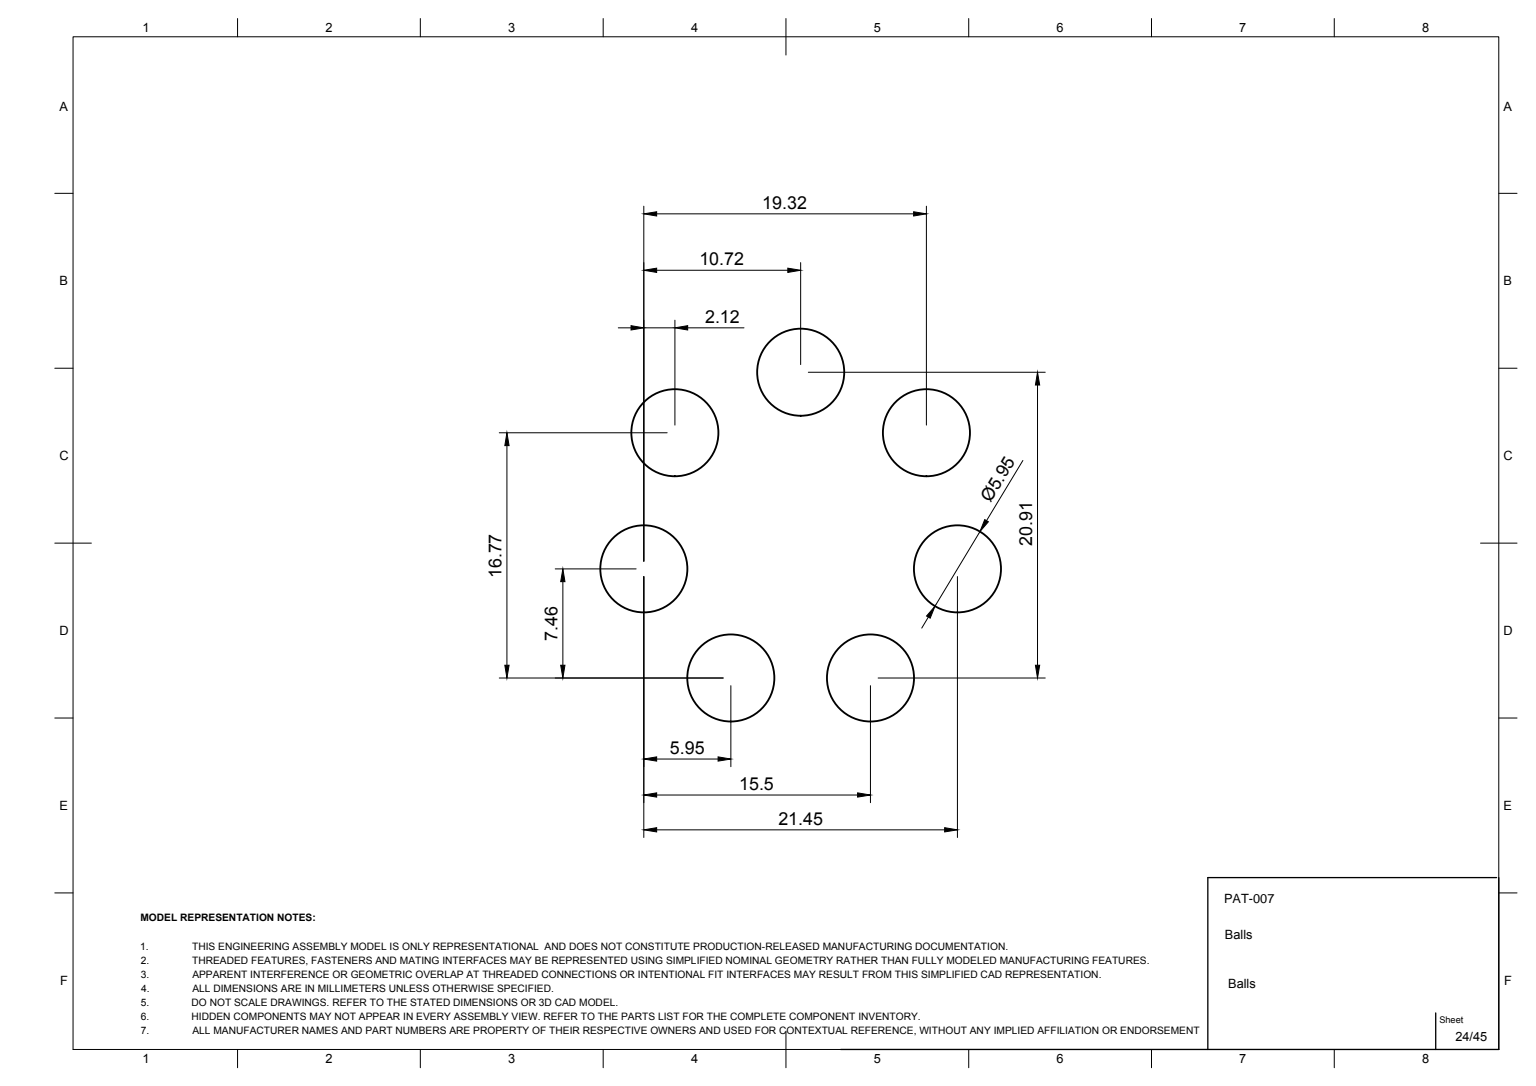
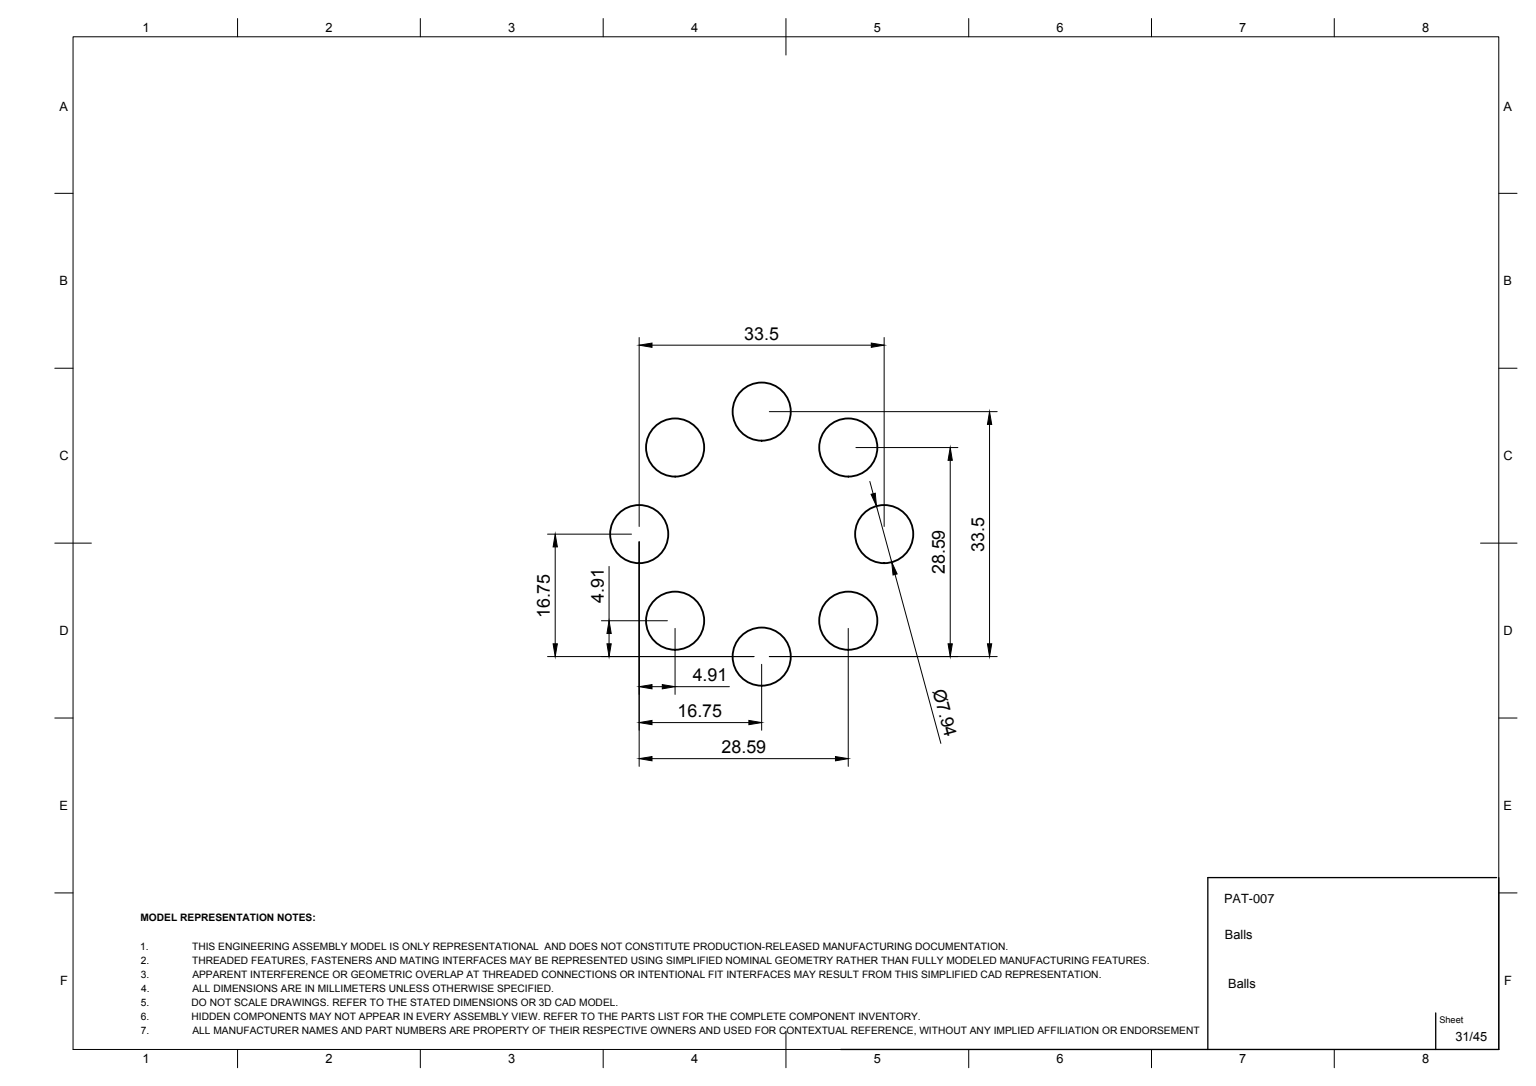
ISO-10303-21;
HEADER;
/* Generated by software containing ST-Developer
 * from STEP Tools, Inc. (www.steptools.com) 
 */

FILE_DESCRIPTION(
/* description */ ('Bearing friction torque test rig'),
/* implementation_level */ '2;1');

FILE_NAME(
/* name */ 'Balls.step',
/* time_stamp */ '2026-10-28T03:24:04-07:00',
/* author */ (''),
/* organization */ (''),
/* preprocessor_version */ 'ST-DEVELOPER v20.2',
/* originating_system */ 'Autodesk Translation Framework v15.17.0.0',
/* authorisation */ '');

FILE_SCHEMA (('AUTOMOTIVE_DESIGN { 1 0 10303 214 3 1 1 }'));
ENDSEC;

DATA;
#10=MECHANICAL_DESIGN_GEOMETRIC_PRESENTATION_REPRESENTATION('',(#557,#558,#559,#560,#561,#562,#563),#14822);
#395=SPHERICAL_SURFACE('',#8664,0.29765);
#396=SPHERICAL_SURFACE('',#8666,0.29765);
#397=SPHERICAL_SURFACE('',#8668,0.29765);
#398=SPHERICAL_SURFACE('',#8670,0.29765);
#399=SPHERICAL_SURFACE('',#8672,0.29765);
#400=SPHERICAL_SURFACE('',#8674,0.29765);
#401=SPHERICAL_SURFACE('',#8676,0.29765);
#479=SHAPE_REPRESENTATION_RELATIONSHIP('SRR','None',#15019,#518);
#518=ADVANCED_BREP_SHAPE_REPRESENTATION('',(#610,#611,#612,#613,#614,#615,
#616),#14799);
#557=STYLED_ITEM('',(#15284),#610);
#558=STYLED_ITEM('',(#15284),#611);
#559=STYLED_ITEM('',(#15284),#612);
#560=STYLED_ITEM('',(#15284),#613);
#561=STYLED_ITEM('',(#15284),#614);
#562=STYLED_ITEM('',(#15284),#615);
#563=STYLED_ITEM('',(#15284),#616);
#610=MANIFOLD_SOLID_BREP('Body1',#7674);
#611=MANIFOLD_SOLID_BREP('Body2',#7675);
#612=MANIFOLD_SOLID_BREP('Body3',#7676);
#613=MANIFOLD_SOLID_BREP('Body4',#7677);
#614=MANIFOLD_SOLID_BREP('Body5',#7678);
#615=MANIFOLD_SOLID_BREP('Body6',#7679);
#616=MANIFOLD_SOLID_BREP('Body7',#7680);
#1352=FACE_OUTER_BOUND('',#1971,.T.);
#1353=FACE_OUTER_BOUND('',#1972,.T.);
#1354=FACE_OUTER_BOUND('',#1973,.T.);
#1355=FACE_OUTER_BOUND('',#1974,.T.);
#1356=FACE_OUTER_BOUND('',#1975,.T.);
#1357=FACE_OUTER_BOUND('',#1976,.T.);
#1358=FACE_OUTER_BOUND('',#1977,.T.);
#1971=EDGE_LOOP('',(#6268,#6269));
#1972=EDGE_LOOP('',(#6270,#6271));
#1973=EDGE_LOOP('',(#6272,#6273));
#1974=EDGE_LOOP('',(#6274,#6275));
#1975=EDGE_LOOP('',(#6276,#6277));
#1976=EDGE_LOOP('',(#6278,#6279));
#1977=EDGE_LOOP('',(#6280,#6281));
#3348=CIRCLE('',#8665,0.29765);
#3349=CIRCLE('',#8667,0.29765);
#3350=CIRCLE('',#8669,0.29765);
#3351=CIRCLE('',#8671,0.29765);
#3352=CIRCLE('',#8673,0.29765);
#3353=CIRCLE('',#8675,0.29765);
#3354=CIRCLE('',#8677,0.29765);
#3924=VERTEX_POINT('',#12865);
#3925=VERTEX_POINT('',#12866);
#3926=VERTEX_POINT('',#12869);
#3927=VERTEX_POINT('',#12870);
#3928=VERTEX_POINT('',#12873);
#3929=VERTEX_POINT('',#12874);
#3930=VERTEX_POINT('',#12877);
#3931=VERTEX_POINT('',#12878);
#3932=VERTEX_POINT('',#12881);
#3933=VERTEX_POINT('',#12882);
#3934=VERTEX_POINT('',#12885);
#3935=VERTEX_POINT('',#12886);
#3936=VERTEX_POINT('',#12889);
#3937=VERTEX_POINT('',#12890);
#4760=EDGE_CURVE('',#3924,#3925,#3348,.T.);
#4761=EDGE_CURVE('',#3926,#3927,#3349,.T.);
#4762=EDGE_CURVE('',#3928,#3929,#3350,.T.);
#4763=EDGE_CURVE('',#3930,#3931,#3351,.T.);
#4764=EDGE_CURVE('',#3932,#3933,#3352,.T.);
#4765=EDGE_CURVE('',#3934,#3935,#3353,.T.);
#4766=EDGE_CURVE('',#3936,#3937,#3354,.T.);
#6268=ORIENTED_EDGE('',*,*,#4760,.T.);
#6269=ORIENTED_EDGE('',*,*,#4760,.F.);
#6270=ORIENTED_EDGE('',*,*,#4761,.T.);
#6271=ORIENTED_EDGE('',*,*,#4761,.F.);
#6272=ORIENTED_EDGE('',*,*,#4762,.T.);
#6273=ORIENTED_EDGE('',*,*,#4762,.F.);
#6274=ORIENTED_EDGE('',*,*,#4763,.T.);
#6275=ORIENTED_EDGE('',*,*,#4763,.F.);
#6276=ORIENTED_EDGE('',*,*,#4764,.T.);
#6277=ORIENTED_EDGE('',*,*,#4764,.F.);
#6278=ORIENTED_EDGE('',*,*,#4765,.T.);
#6279=ORIENTED_EDGE('',*,*,#4765,.F.);
#6280=ORIENTED_EDGE('',*,*,#4766,.T.);
#6281=ORIENTED_EDGE('',*,*,#4766,.F.);
#7463=ADVANCED_FACE('',(#1352),#395,.T.);
#7464=ADVANCED_FACE('',(#1353),#396,.T.);
#7465=ADVANCED_FACE('',(#1354),#397,.T.);
#7466=ADVANCED_FACE('',(#1355),#398,.T.);
#7467=ADVANCED_FACE('',(#1356),#399,.T.);
#7468=ADVANCED_FACE('',(#1357),#400,.T.);
#7469=ADVANCED_FACE('',(#1358),#401,.T.);
#7674=CLOSED_SHELL('',(#7463));
#7675=CLOSED_SHELL('',(#7464));
#7676=CLOSED_SHELL('',(#7465));
#7677=CLOSED_SHELL('',(#7466));
#7678=CLOSED_SHELL('',(#7467));
#7679=CLOSED_SHELL('',(#7468));
#7680=CLOSED_SHELL('',(#7469));
#8663=AXIS2_PLACEMENT_3D('',#12863,#10521,#10522);
#8664=AXIS2_PLACEMENT_3D('',#12864,#10523,#10524);
#8665=AXIS2_PLACEMENT_3D('',#12867,#10525,#10526);
#8666=AXIS2_PLACEMENT_3D('',#12868,#10527,#10528);
#8667=AXIS2_PLACEMENT_3D('',#12871,#10529,#10530);
#8668=AXIS2_PLACEMENT_3D('',#12872,#10531,#10532);
#8669=AXIS2_PLACEMENT_3D('',#12875,#10533,#10534);
#8670=AXIS2_PLACEMENT_3D('',#12876,#10535,#10536);
#8671=AXIS2_PLACEMENT_3D('',#12879,#10537,#10538);
#8672=AXIS2_PLACEMENT_3D('',#12880,#10539,#10540);
#8673=AXIS2_PLACEMENT_3D('',#12883,#10541,#10542);
#8674=AXIS2_PLACEMENT_3D('',#12884,#10543,#10544);
#8675=AXIS2_PLACEMENT_3D('',#12887,#10545,#10546);
#8676=AXIS2_PLACEMENT_3D('',#12888,#10547,#10548);
#8677=AXIS2_PLACEMENT_3D('',#12891,#10549,#10550);
#10521=DIRECTION('axis',(0.,0.,1.));
#10522=DIRECTION('refdir',(1.,0.,0.));
#10523=DIRECTION('center_axis',(0.,0.,1.));
#10524=DIRECTION('ref_axis',(1.,0.,0.));
#10525=DIRECTION('center_axis',(1.22464679914735E-16,-1.,0.));
#10526=DIRECTION('ref_axis',(-1.,-1.22464679914735E-16,0.));
#10527=DIRECTION('center_axis',(0.78183148246803,0.,0.623489801858733));
#10528=DIRECTION('ref_axis',(0.623489801858734,0.,-0.78183148246803));
#10529=DIRECTION('center_axis',(7.63554790147315E-17,-1.,-9.57467422477103E-17));
#10530=DIRECTION('ref_axis',(-0.623489801858734,-1.22464679914735E-16,0.78183148246803));
#10531=DIRECTION('center_axis',(0.974927912181824,0.,-0.222520933956314));
#10532=DIRECTION('ref_axis',(-0.222520933956314,0.,-0.974927912181824));
#10533=DIRECTION('center_axis',(-2.7250954951288E-17,-1.,-1.19394234705288E-16));
#10534=DIRECTION('ref_axis',(0.222520933956314,-1.22464679914735E-16,0.974927912181824));
#10535=DIRECTION('center_axis',(0.433883739117558,0.,-0.900968867902419));
#10536=DIRECTION('ref_axis',(-0.900968867902419,0.,-0.433883739117558));
#10537=DIRECTION('center_axis',(-1.10336864020811E-16,-1.,-5.31354332312403E-17));
#10538=DIRECTION('ref_axis',(0.900968867902419,-1.22464679914735E-16,0.433883739117558));
#10539=DIRECTION('center_axis',(-0.433883739117558,0.,-0.900968867902419));
#10540=DIRECTION('ref_axis',(-0.900968867902419,0.,0.433883739117558));
#10541=DIRECTION('center_axis',(-1.10336864020811E-16,-1.,5.31354332312403E-17));
#10542=DIRECTION('ref_axis',(0.900968867902419,-1.22464679914735E-16,-0.433883739117558));
#10543=DIRECTION('center_axis',(-0.974927912181824,0.,-0.222520933956314));
#10544=DIRECTION('ref_axis',(-0.222520933956315,0.,0.974927912181824));
#10545=DIRECTION('center_axis',(-2.7250954951288E-17,-1.,1.19394234705288E-16));
#10546=DIRECTION('ref_axis',(0.222520933956315,-1.22464679914735E-16,-0.974927912181824));
#10547=DIRECTION('center_axis',(-0.78183148246803,0.,0.623489801858734));
#10548=DIRECTION('ref_axis',(0.623489801858733,0.,0.78183148246803));
#10549=DIRECTION('center_axis',(7.63554790147315E-17,-1.,9.57467422477103E-17));
#10550=DIRECTION('ref_axis',(-0.623489801858733,-1.22464679914735E-16,-0.78183148246803));
#12863=CARTESIAN_POINT('',(0.,0.,0.));
#12864=CARTESIAN_POINT('Origin',(1.1,0.,0.));
#12865=CARTESIAN_POINT('',(1.1,-2.23201749654651E-33,0.29765));
#12866=CARTESIAN_POINT('',(1.1,-2.23201749654651E-33,-0.29765));
#12867=CARTESIAN_POINT('Origin',(1.1,0.,0.));
#12868=CARTESIAN_POINT('Origin',(0.685838782044607,0.,-0.860014630714833));
#12869=CARTESIAN_POINT('',(0.918550922801216,-5.31350540756609E-33,-0.674432891191581));
#12870=CARTESIAN_POINT('',(0.453126641287998,8.49470414473068E-34,-1.04559637023808));
#12871=CARTESIAN_POINT('Origin',(0.685838782044607,0.,-0.860014630714833));
#12872=CARTESIAN_POINT('Origin',(-0.244773027351946,0.,-1.07242070340001));
#12873=CARTESIAN_POINT('',(0.0454142657089739,-2.23201749654651E-33,-1.1386540593921));
#12874=CARTESIAN_POINT('',(-0.534960320412865,-2.23201749654651E-33,-1.00618734740791));
#12875=CARTESIAN_POINT('Origin',(-0.244773027351946,0.,-1.07242070340001));
#12876=CARTESIAN_POINT('Origin',(-0.991065754692661,0.,-0.477272113029314));
#12877=CARTESIAN_POINT('',(-0.86192025974432,8.49470414473067E-34,-0.745445496560469));
#12878=CARTESIAN_POINT('',(-1.120211249641,-5.31350540756609E-33,-0.209098729498159));
#12879=CARTESIAN_POINT('Origin',(-0.991065754692661,0.,-0.477272113029314));
#12880=CARTESIAN_POINT('Origin',(-0.991065754692661,0.,0.477272113029314));
#12881=CARTESIAN_POINT('',(-1.120211249641,-2.23201749654651E-33,0.209098729498159));
#12882=CARTESIAN_POINT('',(-0.86192025974432,-2.23201749654651E-33,0.745445496560469));
#12883=CARTESIAN_POINT('Origin',(-0.991065754692661,0.,0.477272113029314));
#12884=CARTESIAN_POINT('Origin',(-0.244773027351946,0.,1.07242070340001));
#12885=CARTESIAN_POINT('',(-0.534960320412866,-2.23201749654651E-33,1.00618734740791));
#12886=CARTESIAN_POINT('',(0.0454142657089737,-2.23201749654651E-33,1.1386540593921));
#12887=CARTESIAN_POINT('Origin',(-0.244773027351946,0.,1.07242070340001));
#12888=CARTESIAN_POINT('Origin',(0.685838782044607,0.,0.860014630714833));
#12889=CARTESIAN_POINT('',(0.453126641287998,-2.23201749654651E-33,1.04559637023808));
#12890=CARTESIAN_POINT('',(0.918550922801216,-2.23201749654651E-33,0.674432891191581));
#12891=CARTESIAN_POINT('Origin',(0.685838782044607,0.,0.860014630714833));
#14754=UNCERTAINTY_MEASURE_WITH_UNIT(LENGTH_MEASURE(0.001),#14823,
'DISTANCE_ACCURACY_VALUE',
'Maximum model space distance between geometric entities at asserted c
onnectivities');
#14777=UNCERTAINTY_MEASURE_WITH_UNIT(LENGTH_MEASURE(0.001),#14823,
'DISTANCE_ACCURACY_VALUE',
'Maximum model space distance between geometric entities at asserted c
onnectivities');
#14799=(
GEOMETRIC_REPRESENTATION_CONTEXT(3)
GLOBAL_UNCERTAINTY_ASSIGNED_CONTEXT((#14754))
GLOBAL_UNIT_ASSIGNED_CONTEXT((#14823,#14825,#14826))
REPRESENTATION_CONTEXT('','3D')
);
#14822=(
GEOMETRIC_REPRESENTATION_CONTEXT(3)
GLOBAL_UNCERTAINTY_ASSIGNED_CONTEXT((#14777))
GLOBAL_UNIT_ASSIGNED_CONTEXT((#14823,#14825,#14826))
REPRESENTATION_CONTEXT('','3D')
);
#14823=(
LENGTH_UNIT()
NAMED_UNIT(*)
SI_UNIT(.CENTI.,.METRE.)
);
#14825=(
NAMED_UNIT(*)
PLANE_ANGLE_UNIT()
SI_UNIT($,.RADIAN.)
);
#14826=(
NAMED_UNIT(*)
SI_UNIT($,.STERADIAN.)
SOLID_ANGLE_UNIT()
);
#14848=SHAPE_DEFINITION_REPRESENTATION(#14892,#15019);
#14892=PRODUCT_DEFINITION_SHAPE('',$,#15064);
#15019=SHAPE_REPRESENTATION('',(#8663),#14799);
#15042=PRODUCT_DEFINITION_CONTEXT('part definition',#15176,'design');
#15064=PRODUCT_DEFINITION('Balls','Balls',#15108,#15042);
#15108=PRODUCT_DEFINITION_FORMATION('',$,#15199);
#15176=APPLICATION_CONTEXT(
'Core Data for Automotive Mechanical Design Process');
#15177=PRODUCT_CONTEXT('part definition',#15176,'mechanical');
#15199=PRODUCT('Balls','Balls','Balls',(#15177));
#15278=COLOUR_RGB('Grey',0.48,0.52,0.57);
#15279=FILL_AREA_STYLE_COLOUR('',#15278);
#15280=FILL_AREA_STYLE('',(#15279));
#15281=SURFACE_STYLE_FILL_AREA(#15280);
#15282=SURFACE_SIDE_STYLE('',(#15281));
#15283=SURFACE_STYLE_USAGE(.BOTH.,#15282);
#15284=PRESENTATION_STYLE_ASSIGNMENT((#15283));
ENDSEC;
END-ISO-10303-21;
